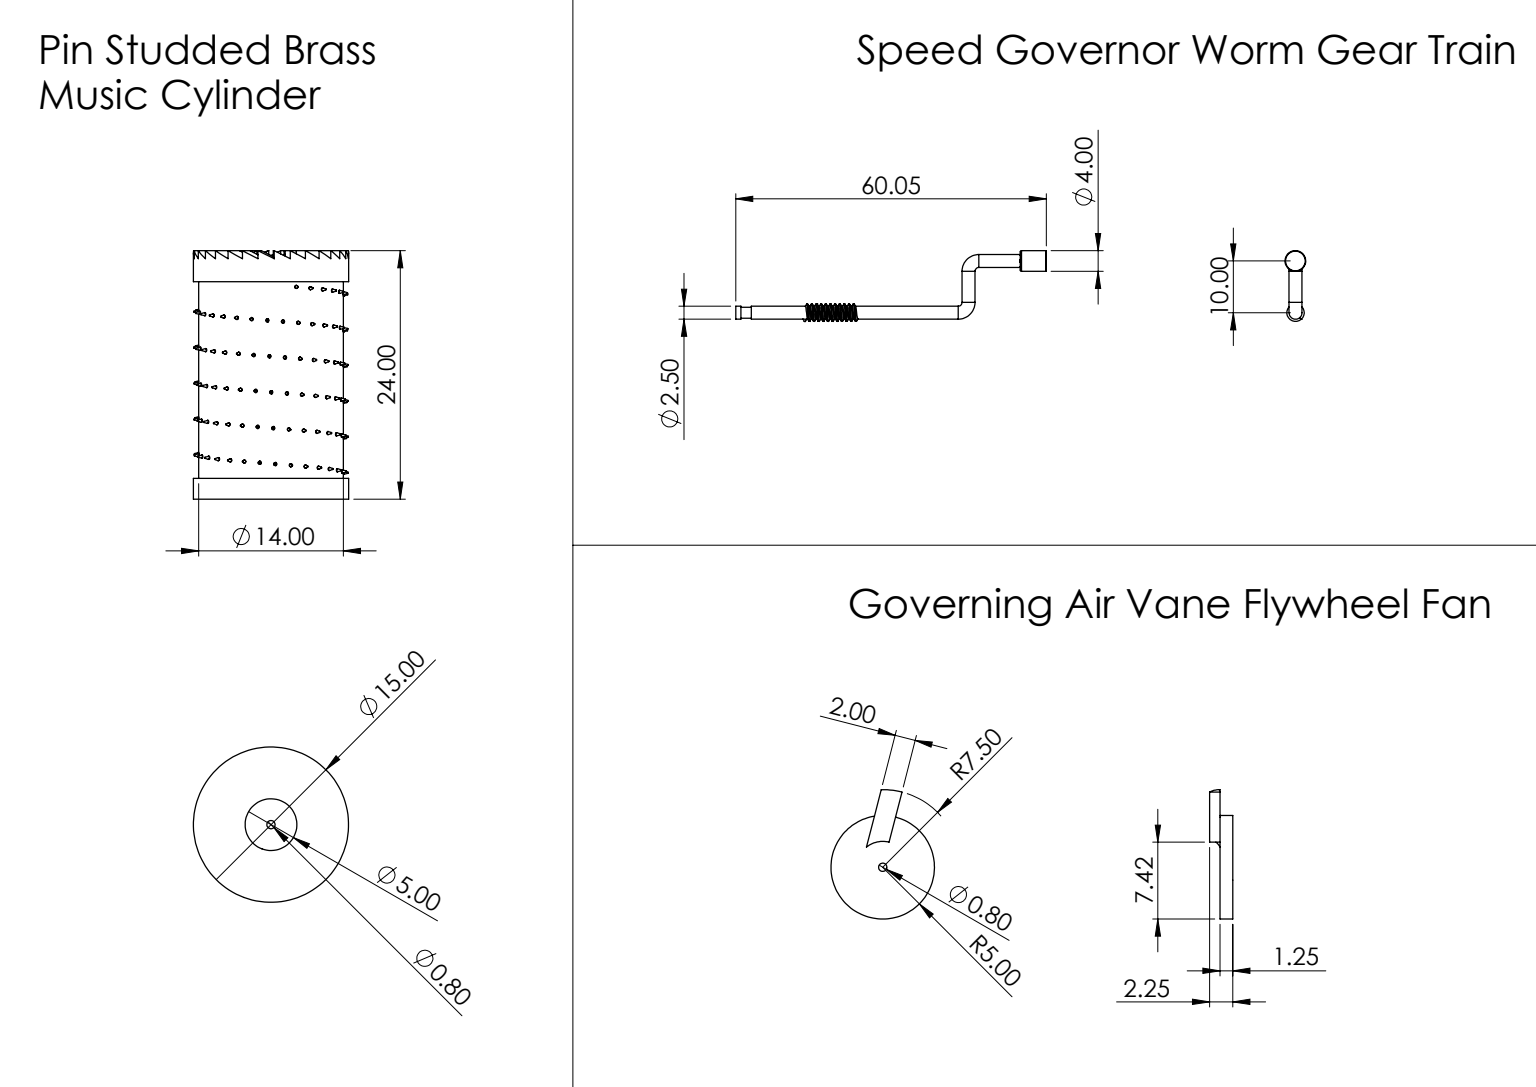
ISO-10303-21;
HEADER;
FILE_DESCRIPTION (('STEP AP214'),
    '1' );
FILE_NAME ('Governing Air Vane Flywheel Fan.step',
    '2026-10-09T09:51:18',
    ( '' ),
    ( '' ),
    'SwSTEP 2.0',
    'SolidWorks 2026',
    '' );
FILE_SCHEMA (( 'AUTOMOTIVE_DESIGN' ));
ENDSEC;

DATA;
#1=SHAPE_REPRESENTATION_RELATIONSHIP ( 'NONE' , 'NONE' ,  #34837, #17929 ) ;
#129=DIRECTION ( 'NONE',  ( 0.9687793358424823253, -0.2479245821708663811, 0.000000000000000000 ) ) ;
#152=MECHANICAL_DESIGN_GEOMETRIC_PRESENTATION_REPRESENTATION('',(#21385),#4091);
#339=PLANE ( 'NONE',  #14810 ) ;
#492=ADVANCED_FACE ( 'NONE', ( #31815, #46833 ), #2013, .F. ) ;
#543=CARTESIAN_POINT ( 'NONE',  ( -17.42409385541300182, -14.80920654474440745, 53.27966884056655061 ) ) ;
#693=ADVANCED_FACE ( 'NONE', ( #1401 ), #695, .F. ) ;
#695=PLANE ( 'NONE',  #46507 ) ;
#898=CIRCLE ( 'NONE', #11896, 7.500000000000000888 ) ;
#1110=ORIENTED_EDGE ( 'NONE', *, *, #21877, .F. ) ;
#1330=CIRCLE ( 'NONE', #8449, 5.000000000000000000 ) ;
#1401=FACE_OUTER_BOUND ( 'NONE', #33780, .T. ) ;
#1613=ORIENTED_EDGE ( 'NONE', *, *, #20351, .F. ) ;
#1939=PRESENTATION_STYLE_ASSIGNMENT (( #10308 ) ) ;
#2013=PLANE ( 'NONE',  #8729 ) ;
#2140=DIRECTION ( 'NONE',  ( 1.702402328345536248E-17, -7.068183862238076217E-18, 1.000000000000000000 ) ) ;
#2668=EDGE_LOOP ( 'NONE', ( #41272, #36699, #13492, #43121 ) ) ;
#3032=CARTESIAN_POINT ( 'NONE',  ( -22.26799053462541522, -13.56958363389006905, 53.27966884056655061 ) ) ;
#3366=VERTEX_POINT ( 'NONE', #36363 ) ;
#3439=ORIENTED_EDGE ( 'NONE', *, *, #5687, .F. ) ;
#3494=CYLINDRICAL_SURFACE ( 'NONE', #31398, 7.500000000000001776 ) ;
#3662=AXIS2_PLACEMENT_3D ( 'NONE', #12276, #35160, #9083 ) ;
#3718=CYLINDRICAL_SURFACE ( 'NONE', #39370, 0.4000000000000011879 ) ;
#3957=VERTEX_POINT ( 'NONE', #14093 ) ;
#3972=DIRECTION ( 'NONE',  ( 3.549360974551883545E-17, -6.371834667872732552E-18, -1.000000000000000000 ) ) ;
#4091=( GEOMETRIC_REPRESENTATION_CONTEXT ( 3 ) GLOBAL_UNCERTAINTY_ASSIGNED_CONTEXT ( ( #6084 ) ) GLOBAL_UNIT_ASSIGNED_CONTEXT ( ( #6365, #25083, #31981 ) ) REPRESENTATION_CONTEXT ( 'NONE', 'WORKASPACE' ) );
#4475=DIRECTION ( 'NONE',  ( -0.9687793358424821033, 0.2479245821708677133, 0.000000000000000000 ) ) ;
#4656=( GEOMETRIC_REPRESENTATION_CONTEXT ( 3 ) GLOBAL_UNCERTAINTY_ASSIGNED_CONTEXT ( ( #23354 ) ) GLOBAL_UNIT_ASSIGNED_CONTEXT ( ( #21908, #18442, #17714 ) ) REPRESENTATION_CONTEXT ( 'NONE', 'WORKASPACE' ) );
#4758=DIRECTION ( 'NONE',  ( 8.136802275736123818E-17, -2.353473986169886338E-17, 1.000000000000000000 ) ) ;
#4797=PRODUCT_DEFINITION_SHAPE ( 'NONE', 'NONE',  #35187 ) ;
#4880=DIRECTION ( 'NONE',  ( 0.4332512900281776380, -0.1108752438054585870, -0.8944271909999159664 ) ) ;
#4890=CARTESIAN_POINT ( 'NONE',  ( -17.42409385541300182, -14.80920654474440745, 53.27966884056655061 ) ) ;
#5179=DIRECTION ( 'NONE',  ( 0.9687793358424821033, -0.2479245821708678243, 0.000000000000000000 ) ) ;
#5204=CARTESIAN_POINT ( 'NONE',  ( -16.80428239998583351, -12.38725820513820253, 54.28066884056654828 ) ) ;
#5239=DIRECTION ( 'NONE',  ( -0.9687793358424821033, 0.2479245821708679631, 8.466249959240414680E-17 ) ) ;
#5346=CYLINDRICAL_SURFACE ( 'NONE', #41841, 2.499999999999999112 ) ;
#5503=CARTESIAN_POINT ( 'NONE',  ( -16.89278889608604572, -7.297489456700872346, 53.60585781316035536 ) ) ;
#5535=VERTEX_POINT ( 'NONE', #27523 ) ;
#5543=CIRCLE ( 'NONE', #25214, 5.000000000000000000 ) ;
#5620=DIRECTION ( 'NONE',  ( 0.9687793358424819923, -0.2479245821708678799, -1.824489850066507969E-17 ) ) ;
#5687=EDGE_CURVE ( 'NONE', #46547, #46160, #30741, .T. ) ;
#5759=DIRECTION ( 'NONE',  ( 3.549360974551883545E-17, -6.371834667872732552E-18, -1.000000000000000000 ) ) ;
#5955=DIRECTION ( 'NONE',  ( 0.9687793358424819923, -0.2479245821708678799, 3.596521012361014201E-17 ) ) ;
#5969=ORIENTED_EDGE ( 'NONE', *, *, #22653, .F. ) ;
#6063=DIRECTION ( 'NONE',  ( -1.702402328345533783E-17, 7.068183862238070054E-18, -1.000000000000000000 ) ) ;
#6084=UNCERTAINTY_MEASURE_WITH_UNIT (LENGTH_MEASURE( 1.000000000000000082E-05 ), #6365, 'distance_accuracy_value', 'NONE');
#6110=CARTESIAN_POINT ( 'NONE',  ( -17.50221816081645798, -7.047512361584055363, 53.27966884056655061 ) ) ;
#6328=CARTESIAN_POINT ( 'NONE',  ( -18.36468646126785842, -12.35805408173462006, 53.52020502545293112 ) ) ;
#6362=ORIENTED_EDGE ( 'NONE', *, *, #8334, .F. ) ;
#6365=( LENGTH_UNIT ( ) NAMED_UNIT ( * ) SI_UNIT ( .MILLI., .METRE. ) );
#6368=CARTESIAN_POINT ( 'NONE',  ( -17.42409385541300182, -14.80920654474440745, 53.27966884056655061 ) ) ;
#6432=VERTEX_POINT ( 'NONE', #37353 ) ;
#6847=DIRECTION ( 'NONE',  ( -3.549360974551883545E-17, 6.371834667872732552E-18, 1.000000000000000000 ) ) ;
#6942=CARTESIAN_POINT ( 'NONE',  ( -15.56465948913149333, -7.543361525925791788, 53.27966884056655061 ) ) ;
#7100=ADVANCED_FACE ( 'NONE', ( #35020 ), #339, .F. ) ;
#7437=ADVANCED_FACE ( 'NONE', ( #12975 ), #16672, .T. ) ;
#7505=ORIENTED_EDGE ( 'NONE', *, *, #10591, .T. ) ;
#7674=FACE_OUTER_BOUND ( 'NONE', #26405, .T. ) ;
#7701=CARTESIAN_POINT ( 'NONE',  ( -17.42409385541300182, -14.80920654474440745, 54.28066884056654828 ) ) ;
#7909=DIRECTION ( 'NONE',  ( -3.549360974551883545E-17, 6.371834667872732552E-18, 1.000000000000000000 ) ) ;
#7974=AXIS2_PLACEMENT_3D ( 'NONE', #6368, #6847, #48206 ) ;
#8005=EDGE_CURVE ( 'NONE', #48120, #46547, #29870, .T. ) ;
#8334=EDGE_CURVE ( 'NONE', #25294, #6432, #42391, .T. ) ;
#8449=AXIS2_PLACEMENT_3D ( 'NONE', #10822, #28815, #36188 ) ;
#8632=VECTOR ( 'NONE', #20706, 1000.000000000000000 ) ;
#8729=AXIS2_PLACEMENT_3D ( 'NONE', #17007, #13080, #5955 ) ;
#9083=DIRECTION ( 'NONE',  ( -0.9687793358424823253, 0.2479245821708663811, 0.000000000000000000 ) ) ;
#9483=LINE ( 'NONE', #3032, #42474 ) ;
#9550=ORIENTED_EDGE ( 'NONE', *, *, #15725, .F. ) ;
#9755=DIRECTION ( 'NONE',  ( -3.549360974551883545E-17, 6.371834667872732552E-18, 1.000000000000000000 ) ) ;
#9925=LINE ( 'NONE', #12644, #15454 ) ;
#10029=ORIENTED_EDGE ( 'NONE', *, *, #23184, .T. ) ;
#10060=SURFACE_STYLE_FILL_AREA ( #16704 ) ;
#10308=SURFACE_STYLE_USAGE ( .BOTH. , #17439 ) ;
#10327=LINE ( 'NONE', #26307, #20963 ) ;
#10554=ADVANCED_FACE ( 'NONE', ( #22970 ), #34259, .T. ) ;
#10591=EDGE_CURVE ( 'NONE', #32748, #46547, #46990, .T. ) ;
#10738=ORIENTED_EDGE ( 'NONE', *, *, #39278, .F. ) ;
#10822=CARTESIAN_POINT ( 'NONE',  ( -17.42409385541300182, -14.80920654474440745, 53.27966884056655061 ) ) ;
#10842=EDGE_LOOP ( 'NONE', ( #6362, #32328, #22768 ) ) ;
#10855=VECTOR ( 'NONE', #17574, 1000.000000000000000 ) ;
#11223=ORIENTED_EDGE ( 'NONE', *, *, #42209, .T. ) ;
#11896=AXIS2_PLACEMENT_3D ( 'NONE', #48152, #6063, #47439 ) ;
#12146=DIRECTION ( 'NONE',  ( -8.136802275736123818E-17, 2.353473986169886647E-17, -1.000000000000000000 ) ) ;
#12276=CARTESIAN_POINT ( 'NONE',  ( -17.42409385541300182, -14.80920654474440745, 53.27966884056655061 ) ) ;
#12375=CARTESIAN_POINT ( 'NONE',  ( -15.56465948913149333, -7.543361525925791788, 53.27966884056655061 ) ) ;
#12644=CARTESIAN_POINT ( 'NONE',  ( -17.81160558974999830, -14.71003671187606088, 53.27966884056655061 ) ) ;
#12711=CARTESIAN_POINT ( 'NONE',  ( -17.42409385541300182, -14.80920654474440745, 53.27966884056655061 ) ) ;
#12726=AXIS2_PLACEMENT_3D ( 'NONE', #22035, #41472, #129 ) ;
#12966=ORIENTED_EDGE ( 'NONE', *, *, #19502, .F. ) ;
#12974=CARTESIAN_POINT ( 'NONE',  ( -18.98976565384166193, -12.86018837663894843, 53.27966884056655061 ) ) ;
#12975=FACE_OUTER_BOUND ( 'NONE', #13840, .T. ) ;
#13007=ORIENTED_EDGE ( 'NONE', *, *, #18349, .T. ) ;
#13067=AXIS2_PLACEMENT_3D ( 'NONE', #43324, #35425, #46537 ) ;
#13080=DIRECTION ( 'NONE',  ( -3.549360974551879847E-17, 6.371834667872723308E-18, 1.000000000000000000 ) ) ;
#13204=CARTESIAN_POINT ( 'NONE',  ( -15.56465948913149155, -7.543361525925791788, 54.27966884056655061 ) ) ;
#13339=CARTESIAN_POINT ( 'NONE',  ( -16.22041545928731310, -7.375544130475720550, 53.94122439512140943 ) ) ;
#13356=ADVANCED_FACE ( 'NONE', ( #38361 ), #30999, .F. ) ;
#13399=CARTESIAN_POINT ( 'NONE',  ( -17.42409385541300182, -14.80920654474440745, 53.27966884056655061 ) ) ;
#13454=PLANE ( 'NONE',  #22403 ) ;
#13482=COLOUR_RGB ( '', 0.09019608, 0.27058824, 0.51372549) ;
#13492=ORIENTED_EDGE ( 'NONE', *, *, #43620, .F. ) ;
#13840=EDGE_LOOP ( 'NONE', ( #44469, #30409, #18958, #1110, #34509, #24882 ) ) ;
#13919=DIRECTION ( 'NONE',  ( -3.549360974551883545E-17, 6.371834667872732552E-18, 1.000000000000000000 ) ) ;
#14093=CARTESIAN_POINT ( 'NONE',  ( -17.03658212107600889, -14.90837637761275403, 53.27966884056655061 ) ) ;
#14129=EDGE_CURVE ( 'NONE', #30553, #37645, #1330, .T. ) ;
#14487=AXIS2_PLACEMENT_3D ( 'NONE', #12711, #9755, #43492 ) ;
#14810=AXIS2_PLACEMENT_3D ( 'NONE', #12375, #5239, #4758 ) ;
#15454=VECTOR ( 'NONE', #5759, 1000.000000000000000 ) ;
#15725=EDGE_CURVE ( 'NONE', #25294, #47754, #16301, .T. ) ;
#16125=ORIENTED_EDGE ( 'NONE', *, *, #20351, .T. ) ;
#16251=CARTESIAN_POINT ( 'NONE',  ( -15.56465948913149333, -7.543361525925791788, 53.27966884056655061 ) ) ;
#16301=LINE ( 'NONE', #38225, #26589 ) ;
#16367=PRODUCT_CONTEXT ( 'NONE', #44189, 'mechanical' ) ;
#16418=DIRECTION ( 'NONE',  ( -0.8665025800563552760, 0.2217504876109172018, -0.4472135954999578722 ) ) ;
#16586=CIRCLE ( 'NONE', #26027, 0.4000000000000011879 ) ;
#16672=CYLINDRICAL_SURFACE ( 'NONE', #48660, 5.000000000000001776 ) ;
#16687=CARTESIAN_POINT ( 'NONE',  ( -17.81160558974999830, -14.71003671187606088, 52.02966884056655061 ) ) ;
#16704=FILL_AREA_STYLE ('',( #28772 ) ) ;
#16882=DIRECTION ( 'NONE',  ( -0.9687793358424821033, 0.2479245821708679076, 0.000000000000000000 ) ) ;
#16996=CIRCLE ( 'NONE', #13067, 5.000000000000000000 ) ;
#17007=CARTESIAN_POINT ( 'NONE',  ( -17.42409385541300182, -14.80920654474440745, 52.02966884056655061 ) ) ;
#17098=ORIENTED_EDGE ( 'NONE', *, *, #19502, .T. ) ;
#17186=ADVANCED_FACE ( 'NONE', ( #21972 ), #3494, .T. ) ;
#17439=SURFACE_SIDE_STYLE ('',( #10060 ) ) ;
#17574=DIRECTION ( 'NONE',  ( 3.549360974551883545E-17, -6.371834667872732552E-18, -1.000000000000000000 ) ) ;
#17714=( NAMED_UNIT ( * ) SI_UNIT ( $, .STERADIAN. ) SOLID_ANGLE_UNIT ( ) );
#17897=ORIENTED_EDGE ( 'NONE', *, *, #30353, .F. ) ;
#17929=ADVANCED_BREP_SHAPE_REPRESENTATION ( '', ( #32222, #29031 ), #4656 ) ;
#18349=EDGE_CURVE ( 'NONE', #46160, #48120, #32278, .T. ) ;
#18413=DIRECTION ( 'NONE',  ( -0.2479245821708678799, -0.9687793358424819923, -2.626836608253746575E-18 ) ) ;
#18442=( NAMED_UNIT ( * ) PLANE_ANGLE_UNIT ( ) SI_UNIT ( $, .RADIAN. ) );
#18637=VERTEX_POINT ( 'NONE', #16687 ) ;
#18709=CARTESIAN_POINT ( 'NONE',  ( -17.42409385541300182, -14.80920654474440745, 52.02966884056655061 ) ) ;
#18723=DIRECTION ( 'NONE',  ( 3.549360974551883545E-17, -6.371834667872732552E-18, -1.000000000000000000 ) ) ;
#18779=FACE_BOUND ( 'NONE', #26205, .T. ) ;
#18958=ORIENTED_EDGE ( 'NONE', *, *, #45705, .T. ) ;
#19061=CARTESIAN_POINT ( 'NONE',  ( -16.18447094455866164, -9.965309865531997602, 53.27966884056655061 ) ) ;
#19342=SHAPE_DEFINITION_REPRESENTATION ( #4797, #34837 ) ;
#19502=EDGE_CURVE ( 'NONE', #40722, #5535, #5543, .T. ) ;
#19771=AXIS2_PLACEMENT_3D ( 'NONE', #36990, #29622, #30128 ) ;
#19833=CARTESIAN_POINT ( 'NONE',  ( -17.81160558974999830, -14.71003671187606088, 53.27966884056655061 ) ) ;
#20351=EDGE_CURVE ( 'NONE', #27679, #30553, #47255, .T. ) ;
#20479=EDGE_CURVE ( 'NONE', #3957, #23794, #16586, .T. ) ;
#20508=CARTESIAN_POINT ( 'NONE',  ( -15.56465948913149155, -7.543361525925791788, 54.27966884056655061 ) ) ;
#20610=CARTESIAN_POINT ( 'NONE',  ( -17.42409385541300182, -14.80920654474440745, 54.28066884056654828 ) ) ;
#20706=DIRECTION ( 'NONE',  ( 3.549360974551883545E-17, -6.371834667872732552E-18, -1.000000000000000000 ) ) ;
#20805=CARTESIAN_POINT ( 'NONE',  ( -17.03658212107600889, -14.90837637761275403, 53.27966884056655061 ) ) ;
#20854=EDGE_LOOP ( 'NONE', ( #30580, #40606, #36536, #16125, #38028, #11223 ) ) ;
#20963=VECTOR ( 'NONE', #18413, 1000.000000000000114 ) ;
#20993=CARTESIAN_POINT ( 'NONE',  ( -15.56465948913149155, -7.543361525925791788, 54.27966884056655061 ) ) ;
#21040=ADVANCED_FACE ( 'NONE', ( #22479, #18779 ), #33530, .T. ) ;
#21109=LINE ( 'NONE', #13204, #45200 ) ;
#21171=PRODUCT_DEFINITION_FORMATION_WITH_SPECIFIED_SOURCE ( 'ANY', '', #33418, .NOT_KNOWN. ) ;
#21268=ORIENTED_EDGE ( 'NONE', *, *, #26392, .T. ) ;
#21271=CLOSED_SHELL ( 'NONE', ( #7437, #13356, #693, #7100, #39212, #21040, #28639, #10554, #492, #17186, #32599 ) ) ;
#21297=ORIENTED_EDGE ( 'NONE', *, *, #42209, .F. ) ;
#21301=CARTESIAN_POINT ( 'NONE',  ( -17.42409385541300182, -14.80920654474440745, 52.02966884056655061 ) ) ;
#21385=STYLED_ITEM ( 'NONE', ( #1939 ), #32222 ) ;
#21485=CARTESIAN_POINT ( 'NONE',  ( -17.56955047399654646, -7.310617185930959216, 53.27966884056655061 ) ) ;
#21498=EDGE_CURVE ( 'NONE', #6432, #47754, #898, .T. ) ;
#21801=ORIENTED_EDGE ( 'NONE', *, *, #42705, .T. ) ;
#21860=LINE ( 'NONE', #36860, #24102 ) ;
#21877=EDGE_CURVE ( 'NONE', #27679, #40722, #9483, .T. ) ;
#21908=( LENGTH_UNIT ( ) NAMED_UNIT ( * ) SI_UNIT ( .MILLI., .METRE. ) );
#21959=DIRECTION ( 'NONE',  ( -0.2479245821708678799, -0.9687793358424819923, -2.626836608253746575E-18 ) ) ;
#21972=FACE_OUTER_BOUND ( 'NONE', #10842, .T. ) ;
#22035=CARTESIAN_POINT ( 'NONE',  ( -17.42409385541300182, -14.80920654474440745, 52.02966884056655061 ) ) ;
#22370=ORIENTED_EDGE ( 'NONE', *, *, #39278, .T. ) ;
#22403=AXIS2_PLACEMENT_3D ( 'NONE', #27765, #2140, #5620 ) ;
#22462=DIRECTION ( 'NONE',  ( -0.9687793358424819923, 0.2479245821708677688, 0.000000000000000000 ) ) ;
#22479=FACE_OUTER_BOUND ( 'NONE', #20854, .T. ) ;
#22653=EDGE_CURVE ( 'NONE', #6432, #32748, #10327, .T. ) ;
#22759=CARTESIAN_POINT ( 'NONE',  ( -16.80428239998583351, -12.38725820513820253, 54.27966884056655061 ) ) ;
#22768=ORIENTED_EDGE ( 'NONE', *, *, #21498, .F. ) ;
#22970=FACE_OUTER_BOUND ( 'NONE', #46291, .T. ) ;
#23184=EDGE_CURVE ( 'NONE', #37645, #32748, #16996, .T. ) ;
#23354=UNCERTAINTY_MEASURE_WITH_UNIT (LENGTH_MEASURE( 1.000000000000000082E-05 ), #21908, 'distance_accuracy_value', 'NONE');
#23373=ORIENTED_EDGE ( 'NONE', *, *, #8005, .F. ) ;
#23390=CIRCLE ( 'NONE', #31257, 0.4000000000000011879 ) ;
#23435=ORIENTED_EDGE ( 'NONE', *, *, #45705, .F. ) ;
#23794=VERTEX_POINT ( 'NONE', #19833 ) ;
#23899=CARTESIAN_POINT ( 'NONE',  ( -17.42409385541300182, -14.80920654474440745, 53.27966884056655061 ) ) ;
#24102=VECTOR ( 'NONE', #44524, 1000.000000000000114 ) ;
#24173=EDGE_LOOP ( 'NONE', ( #33622, #21268, #10029, #5969 ) ) ;
#24265=LINE ( 'NONE', #20805, #10855 ) ;
#24312=CARTESIAN_POINT ( 'NONE',  ( -12.58019717620059197, -16.04882945559874585, 53.27966884056655061 ) ) ;
#24507=DIRECTION ( 'NONE',  ( 3.549360974551883545E-17, -6.371834667872732552E-18, -1.000000000000000000 ) ) ;
#24832=EDGE_CURVE ( 'NONE', #3957, #3366, #24265, .T. ) ;
#24882=ORIENTED_EDGE ( 'NONE', *, *, #23184, .F. ) ;
#25083=( NAMED_UNIT ( * ) PLANE_ANGLE_UNIT ( ) SI_UNIT ( $, .RADIAN. ) );
#25214=AXIS2_PLACEMENT_3D ( 'NONE', #36720, #29125, #47116 ) ;
#25294=VERTEX_POINT ( 'NONE', #20508 ) ;
#25440=ORIENTED_EDGE ( 'NONE', *, *, #43620, .T. ) ;
#25444=CIRCLE ( 'NONE', #38825, 5.000000000000000000 ) ;
#25864=VECTOR ( 'NONE', #21959, 1000.000000000000114 ) ;
#25948=ORIENTED_EDGE ( 'NONE', *, *, #38732, .F. ) ;
#26027=AXIS2_PLACEMENT_3D ( 'NONE', #29748, #29996, #45031 ) ;
#26205=EDGE_LOOP ( 'NONE', ( #25948, #38342 ) ) ;
#26307=CARTESIAN_POINT ( 'NONE',  ( -17.50221816081645798, -7.047512361584055363, 53.27966884056655061 ) ) ;
#26392=EDGE_CURVE ( 'NONE', #47754, #37645, #32789, .T. ) ;
#26405=EDGE_LOOP ( 'NONE', ( #41155, #47169, #21801, #17897 ) ) ;
#26589=VECTOR ( 'NONE', #12146, 1000.000000000000000 ) ;
#26879=CARTESIAN_POINT ( 'NONE',  ( -18.98976565384166193, -12.86018837663894843, 53.27966884056655061 ) ) ;
#27024=ORIENTED_EDGE ( 'NONE', *, *, #22653, .T. ) ;
#27523=CARTESIAN_POINT ( 'NONE',  ( -12.58019717620059197, -16.04882945559874585, 52.02966884056655061 ) ) ;
#27679=VERTEX_POINT ( 'NONE', #27810 ) ;
#27744=ORIENTED_EDGE ( 'NONE', *, *, #26392, .F. ) ;
#27765=CARTESIAN_POINT ( 'NONE',  ( -17.50221816081645798, -7.047512361584055363, 53.27966884056655061 ) ) ;
#27810=CARTESIAN_POINT ( 'NONE',  ( -22.26799053462541522, -13.56958363389006905, 53.27966884056655061 ) ) ;
#27916=EDGE_LOOP ( 'NONE', ( #23373, #33754, #3439 ) ) ;
#28000=CARTESIAN_POINT ( 'NONE',  ( -17.58103735145357760, -12.18847542802175532, 53.87877519908923318 ) ) ;
#28287=AXIS2_PLACEMENT_3D ( 'NONE', #13399, #47407, #36052 ) ;
#28479=FACE_OUTER_BOUND ( 'NONE', #27916, .T. ) ;
#28639=ADVANCED_FACE ( 'NONE', ( #7674 ), #3718, .F. ) ;
#28772=FILL_AREA_STYLE_COLOUR ( '', #13482 ) ;
#28815=DIRECTION ( 'NONE',  ( -3.549360974551883545E-17, 6.371834667872732552E-18, 1.000000000000000000 ) ) ;
#29031=AXIS2_PLACEMENT_3D ( 'NONE', #29301, #44568, #33698 ) ;
#29125=DIRECTION ( 'NONE',  ( -3.549360974551883545E-17, 6.371834667872732552E-18, 1.000000000000000000 ) ) ;
#29248=CIRCLE ( 'NONE', #12726, 0.4000000000000011879 ) ;
#29301=CARTESIAN_POINT ( 'NONE',  ( 0.000000000000000000, 0.000000000000000000, 0.000000000000000000 ) ) ;
#29540=CARTESIAN_POINT ( 'NONE',  ( -22.26799053462541522, -13.56958363389006905, 52.02966884056655061 ) ) ;
#29622=DIRECTION ( 'NONE',  ( -3.549360974551879847E-17, 6.371834667872723308E-18, 1.000000000000000000 ) ) ;
#29679=CARTESIAN_POINT ( 'NONE',  ( -18.22551936265966432, -9.873852742195451171, 53.27966884056655061 ) ) ;
#29748=CARTESIAN_POINT ( 'NONE',  ( -17.42409385541300182, -14.80920654474440745, 53.27966884056655061 ) ) ;
#29814=DIRECTION ( 'NONE',  ( 0.9687793358424823253, -0.2479245821708663811, 0.000000000000000000 ) ) ;
#29870=CIRCLE ( 'NONE', #28287, 2.499999999999999112 ) ;
#29996=DIRECTION ( 'NONE',  ( -3.549360974551883545E-17, 6.371834667872732552E-18, 1.000000000000000000 ) ) ;
#30128=DIRECTION ( 'NONE',  ( 0.9687793358424819923, -0.2479245821708678799, 3.596521012361014201E-17 ) ) ;
#30353=EDGE_CURVE ( 'NONE', #3366, #18637, #29248, .T. ) ;
#30409=ORIENTED_EDGE ( 'NONE', *, *, #36438, .T. ) ;
#30553=VERTEX_POINT ( 'NONE', #38991 ) ;
#30580=ORIENTED_EDGE ( 'NONE', *, *, #8005, .T. ) ;
#30741=( BOUNDED_CURVE ( )  B_SPLINE_CURVE ( 3, ( #12974, #6328, #28000, #48170 ),
 .UNSPECIFIED., .F., .F. ) 
 B_SPLINE_CURVE_WITH_KNOTS ( ( 4, 4 ),
 ( 0.6435011087932844820, 1.570796326794896558 ),
 .UNSPECIFIED. ) 
 CURVE ( )  GEOMETRIC_REPRESENTATION_ITEM ( )  RATIONAL_B_SPLINE_CURVE ( ( 1.000000000000000000, 0.9296181273332770889, 0.9296181273332770889, 1.000000000000000000 ) ) 
 REPRESENTATION_ITEM ( '' )  );
#30999=CYLINDRICAL_SURFACE ( 'NONE', #3662, 0.4000000000000011879 ) ;
#31065=EDGE_LOOP ( 'NONE', ( #12966, #23435 ) ) ;
#31257=AXIS2_PLACEMENT_3D ( 'NONE', #18709, #7909, #29814 ) ;
#31398=AXIS2_PLACEMENT_3D ( 'NONE', #7701, #48554, #22462 ) ;
#31815=FACE_BOUND ( 'NONE', #36263, .T. ) ;
#31981=( NAMED_UNIT ( * ) SI_UNIT ( $, .STERADIAN. ) SOLID_ANGLE_UNIT ( ) );
#32222=MANIFOLD_SOLID_BREP ( 'Stock-MAS-175-1', #21271 ) ;
#32278=LINE ( 'NONE', #5204, #8632 ) ;
#32328=ORIENTED_EDGE ( 'NONE', *, *, #15725, .T. ) ;
#32599=ADVANCED_FACE ( 'NONE', ( #28479 ), #5346, .F. ) ;
#32748=VERTEX_POINT ( 'NONE', #29679 ) ;
#32789=LINE ( 'NONE', #6942, #25864 ) ;
#33418=PRODUCT ( 'Governing Air Vane Flywheel Fan', 'Governing Air Vane Flywheel Fan', '', ( #16367 ) ) ;
#33518=ORIENTED_EDGE ( 'NONE', *, *, #36438, .F. ) ;
#33530=PLANE ( 'NONE',  #19771 ) ;
#33622=ORIENTED_EDGE ( 'NONE', *, *, #21498, .T. ) ;
#33698=DIRECTION ( 'NONE',  ( 1.000000000000000000, 0.000000000000000000, 0.000000000000000000 ) ) ;
#33754=ORIENTED_EDGE ( 'NONE', *, *, #18349, .F. ) ;
#33780=EDGE_LOOP ( 'NONE', ( #40937, #10738, #40757, #27024, #7505 ) ) ;
#34127=EDGE_CURVE ( 'NONE', #32748, #27679, #25444, .T. ) ;
#34259=CYLINDRICAL_SURFACE ( 'NONE', #42567, 5.000000000000001776 ) ;
#34399=CARTESIAN_POINT ( 'NONE',  ( -15.56465948913149155, -7.543361525925791788, 54.27966884056655061 ) ) ;
#34472=DIRECTION ( 'NONE',  ( -0.9687793358424823253, 0.2479245821708663811, 0.000000000000000000 ) ) ;
#34509=ORIENTED_EDGE ( 'NONE', *, *, #34127, .F. ) ;
#34837=SHAPE_REPRESENTATION ( 'Governing Air Vane Flywheel Fan', ( #29031 ), #4656 ) ;
#35020=FACE_OUTER_BOUND ( 'NONE', #47984, .T. ) ;
#35160=DIRECTION ( 'NONE',  ( 3.549360974551883545E-17, -6.371834667872732552E-18, -1.000000000000000000 ) ) ;
#35187=PRODUCT_DEFINITION ( 'UNKNOWN', '', #21171, #39578 ) ;
#35425=DIRECTION ( 'NONE',  ( -3.549360974551883545E-17, 6.371834667872732552E-18, 1.000000000000000000 ) ) ;
#35604=DIRECTION ( 'NONE',  ( 3.549360974551883545E-17, -6.371834667872732552E-18, -1.000000000000000000 ) ) ;
#36052=DIRECTION ( 'NONE',  ( 0.9687793358424821033, -0.2479245821708679076, 0.000000000000000000 ) ) ;
#36105=DIRECTION ( 'NONE',  ( -0.2479245821708678799, -0.9687793358424819923, -2.626836608253746575E-18 ) ) ;
#36188=DIRECTION ( 'NONE',  ( 0.9687793358424821033, -0.2479245821708678243, 0.000000000000000000 ) ) ;
#36263=EDGE_LOOP ( 'NONE', ( #25440, #48647 ) ) ;
#36363=CARTESIAN_POINT ( 'NONE',  ( -17.03658212107600889, -14.90837637761275403, 52.02966884056655061 ) ) ;
#36438=EDGE_CURVE ( 'NONE', #30553, #5535, #43011, .T. ) ;
#36536=ORIENTED_EDGE ( 'NONE', *, *, #34127, .T. ) ;
#36699=ORIENTED_EDGE ( 'NONE', *, *, #24832, .T. ) ;
#36720=CARTESIAN_POINT ( 'NONE',  ( -17.42409385541300182, -14.80920654474440745, 52.02966884056655061 ) ) ;
#36860=CARTESIAN_POINT ( 'NONE',  ( -15.56465948913149333, -7.543361525925791788, 53.27966884056655061 ) ) ;
#36990=CARTESIAN_POINT ( 'NONE',  ( -17.42409385541300182, -14.80920654474440745, 53.27966884056655061 ) ) ;
#37353=CARTESIAN_POINT ( 'NONE',  ( -17.56955047399654646, -7.310617185930959216, 53.27966884056655061 ) ) ;
#37423=CARTESIAN_POINT ( 'NONE',  ( -17.42409385541300182, -14.80920654474440745, 53.27966884056655061 ) ) ;
#37645=VERTEX_POINT ( 'NONE', #19061 ) ;
#38008=ORIENTED_EDGE ( 'NONE', *, *, #21877, .T. ) ;
#38028=ORIENTED_EDGE ( 'NONE', *, *, #14129, .T. ) ;
#38110=VECTOR ( 'NONE', #39318, 1000.000000000000000 ) ;
#38193=DIRECTION ( 'NONE',  ( 3.549360974551883545E-17, -6.371834667872732552E-18, -1.000000000000000000 ) ) ;
#38225=CARTESIAN_POINT ( 'NONE',  ( -15.56465948913149333, -7.543361525925791788, 53.27966884056655061 ) ) ;
#38342=ORIENTED_EDGE ( 'NONE', *, *, #20479, .F. ) ;
#38361=FACE_OUTER_BOUND ( 'NONE', #2668, .T. ) ;
#38732=EDGE_CURVE ( 'NONE', #23794, #3957, #40461, .T. ) ;
#38825=AXIS2_PLACEMENT_3D ( 'NONE', #23899, #13919, #5179 ) ;
#38991=CARTESIAN_POINT ( 'NONE',  ( -12.58019717620059197, -16.04882945559874585, 53.27966884056655061 ) ) ;
#39119=APPLICATION_CONTEXT ( 'automotive_design' ) ;
#39212=ADVANCED_FACE ( 'NONE', ( #39572 ), #13454, .F. ) ;
#39278=EDGE_CURVE ( 'NONE', #25294, #46160, #21109, .T. ) ;
#39318=DIRECTION ( 'NONE',  ( 3.549360974551883545E-17, -6.371834667872732552E-18, -1.000000000000000000 ) ) ;
#39364=DIRECTION ( 'NONE',  ( -0.2479245821708678799, -0.9687793358424819923, -2.626836608253746575E-18 ) ) ;
#39370=AXIS2_PLACEMENT_3D ( 'NONE', #37423, #18723, #34472 ) ;
#39572=FACE_OUTER_BOUND ( 'NONE', #24173, .T. ) ;
#39578=PRODUCT_DEFINITION_CONTEXT ( 'detailed design', #39119, 'design' ) ;
#40461=CIRCLE ( 'NONE', #14487, 0.4000000000000011879 ) ;
#40606=ORIENTED_EDGE ( 'NONE', *, *, #10591, .F. ) ;
#40722=VERTEX_POINT ( 'NONE', #29540 ) ;
#40741=AXIS2_PLACEMENT_3D ( 'NONE', #21301, #42973, #47405 ) ;
#40757=ORIENTED_EDGE ( 'NONE', *, *, #8334, .T. ) ;
#40937=ORIENTED_EDGE ( 'NONE', *, *, #5687, .T. ) ;
#40963=VECTOR ( 'NONE', #39364, 1000.000000000000114 ) ;
#41155=ORIENTED_EDGE ( 'NONE', *, *, #24832, .F. ) ;
#41272=ORIENTED_EDGE ( 'NONE', *, *, #38732, .T. ) ;
#41472=DIRECTION ( 'NONE',  ( -3.549360974551883545E-17, 6.371834667872732552E-18, 1.000000000000000000 ) ) ;
#41841=AXIS2_PLACEMENT_3D ( 'NONE', #20610, #35604, #16882 ) ;
#42209=EDGE_CURVE ( 'NONE', #37645, #48120, #21860, .T. ) ;
#42391=( BOUNDED_CURVE ( )  B_SPLINE_CURVE ( 3, ( #20993, #13339, #5503, #21485 ),
 .UNSPECIFIED., .F., .F. ) 
 B_SPLINE_CURVE_WITH_KNOTS ( ( 4, 4 ),
 ( 4.712388980384689674, 4.982321776218093135 ),
 .UNSPECIFIED. ) 
 CURVE ( )  GEOMETRIC_REPRESENTATION_ITEM ( )  RATIONAL_B_SPLINE_CURVE ( ( 1.000000000000000000, 0.9939372354399834686, 0.9939372354399834686, 1.000000000000000000 ) ) 
 REPRESENTATION_ITEM ( '' )  );
#42474=VECTOR ( 'NONE', #24507, 1000.000000000000000 ) ;
#42567=AXIS2_PLACEMENT_3D ( 'NONE', #543, #38193, #4475 ) ;
#42705=EDGE_CURVE ( 'NONE', #23794, #18637, #9925, .T. ) ;
#42973=DIRECTION ( 'NONE',  ( -3.549360974551883545E-17, 6.371834667872732552E-18, 1.000000000000000000 ) ) ;
#43011=LINE ( 'NONE', #24312, #38110 ) ;
#43028=DIRECTION ( 'NONE',  ( -0.9687793358424821033, 0.2479245821708677133, 0.000000000000000000 ) ) ;
#43111=CIRCLE ( 'NONE', #40741, 5.000000000000000000 ) ;
#43121=ORIENTED_EDGE ( 'NONE', *, *, #42705, .F. ) ;
#43324=CARTESIAN_POINT ( 'NONE',  ( -17.42409385541300182, -14.80920654474440745, 53.27966884056655061 ) ) ;
#43492=DIRECTION ( 'NONE',  ( 0.9687793358424823253, -0.2479245821708663811, 0.000000000000000000 ) ) ;
#43620=EDGE_CURVE ( 'NONE', #18637, #3366, #23390, .T. ) ;
#44189=APPLICATION_CONTEXT ( 'automotive_design' ) ;
#44469=ORIENTED_EDGE ( 'NONE', *, *, #14129, .F. ) ;
#44524=DIRECTION ( 'NONE',  ( -0.2479245821708678799, -0.9687793358424819923, -2.626836608253746575E-18 ) ) ;
#44568=DIRECTION ( 'NONE',  ( 0.000000000000000000, 0.000000000000000000, 1.000000000000000000 ) ) ;
#45031=DIRECTION ( 'NONE',  ( 0.9687793358424823253, -0.2479245821708663811, 0.000000000000000000 ) ) ;
#45200=VECTOR ( 'NONE', #36105, 1000.000000000000114 ) ;
#45705=EDGE_CURVE ( 'NONE', #5535, #40722, #43111, .T. ) ;
#46160=VERTEX_POINT ( 'NONE', #22759 ) ;
#46291=EDGE_LOOP ( 'NONE', ( #33518, #1613, #38008, #17098 ) ) ;
#46507=AXIS2_PLACEMENT_3D ( 'NONE', #34399, #4880, #16418 ) ;
#46537=DIRECTION ( 'NONE',  ( 0.9687793358424821033, -0.2479245821708678243, 0.000000000000000000 ) ) ;
#46547=VERTEX_POINT ( 'NONE', #26879 ) ;
#46833=FACE_OUTER_BOUND ( 'NONE', #31065, .T. ) ;
#46990=LINE ( 'NONE', #6110, #40963 ) ;
#47116=DIRECTION ( 'NONE',  ( 0.9687793358424821033, -0.2479245821708678243, 0.000000000000000000 ) ) ;
#47169=ORIENTED_EDGE ( 'NONE', *, *, #20479, .T. ) ;
#47255=CIRCLE ( 'NONE', #7974, 5.000000000000000000 ) ;
#47405=DIRECTION ( 'NONE',  ( 0.9687793358424821033, -0.2479245821708678243, 0.000000000000000000 ) ) ;
#47407=DIRECTION ( 'NONE',  ( -3.549360974551883545E-17, 6.371834667872732552E-18, 1.000000000000000000 ) ) ;
#47439=DIRECTION ( 'NONE',  ( 0.9687793358424811041, -0.2479245821708714881, 0.000000000000000000 ) ) ;
#47754=VERTEX_POINT ( 'NONE', #16251 ) ;
#47984=EDGE_LOOP ( 'NONE', ( #13007, #21297, #27744, #9550, #22370 ) ) ;
#48120=VERTEX_POINT ( 'NONE', #48185 ) ;
#48152=CARTESIAN_POINT ( 'NONE',  ( -17.42409385541300182, -14.80920654474440745, 53.27966884056655061 ) ) ;
#48170=CARTESIAN_POINT ( 'NONE',  ( -16.80428239998583351, -12.38725820513820253, 54.27966884056655061 ) ) ;
#48185=CARTESIAN_POINT ( 'NONE',  ( -16.80428239998583351, -12.38725820513820253, 53.27966884056655061 ) ) ;
#48206=DIRECTION ( 'NONE',  ( 0.9687793358424821033, -0.2479245821708678243, 0.000000000000000000 ) ) ;
#48554=DIRECTION ( 'NONE',  ( 3.549360974551883545E-17, -6.371834667872732552E-18, -1.000000000000000000 ) ) ;
#48647=ORIENTED_EDGE ( 'NONE', *, *, #30353, .T. ) ;
#48660=AXIS2_PLACEMENT_3D ( 'NONE', #4890, #3972, #43028 ) ;
ENDSEC;
END-ISO-10303-21;
